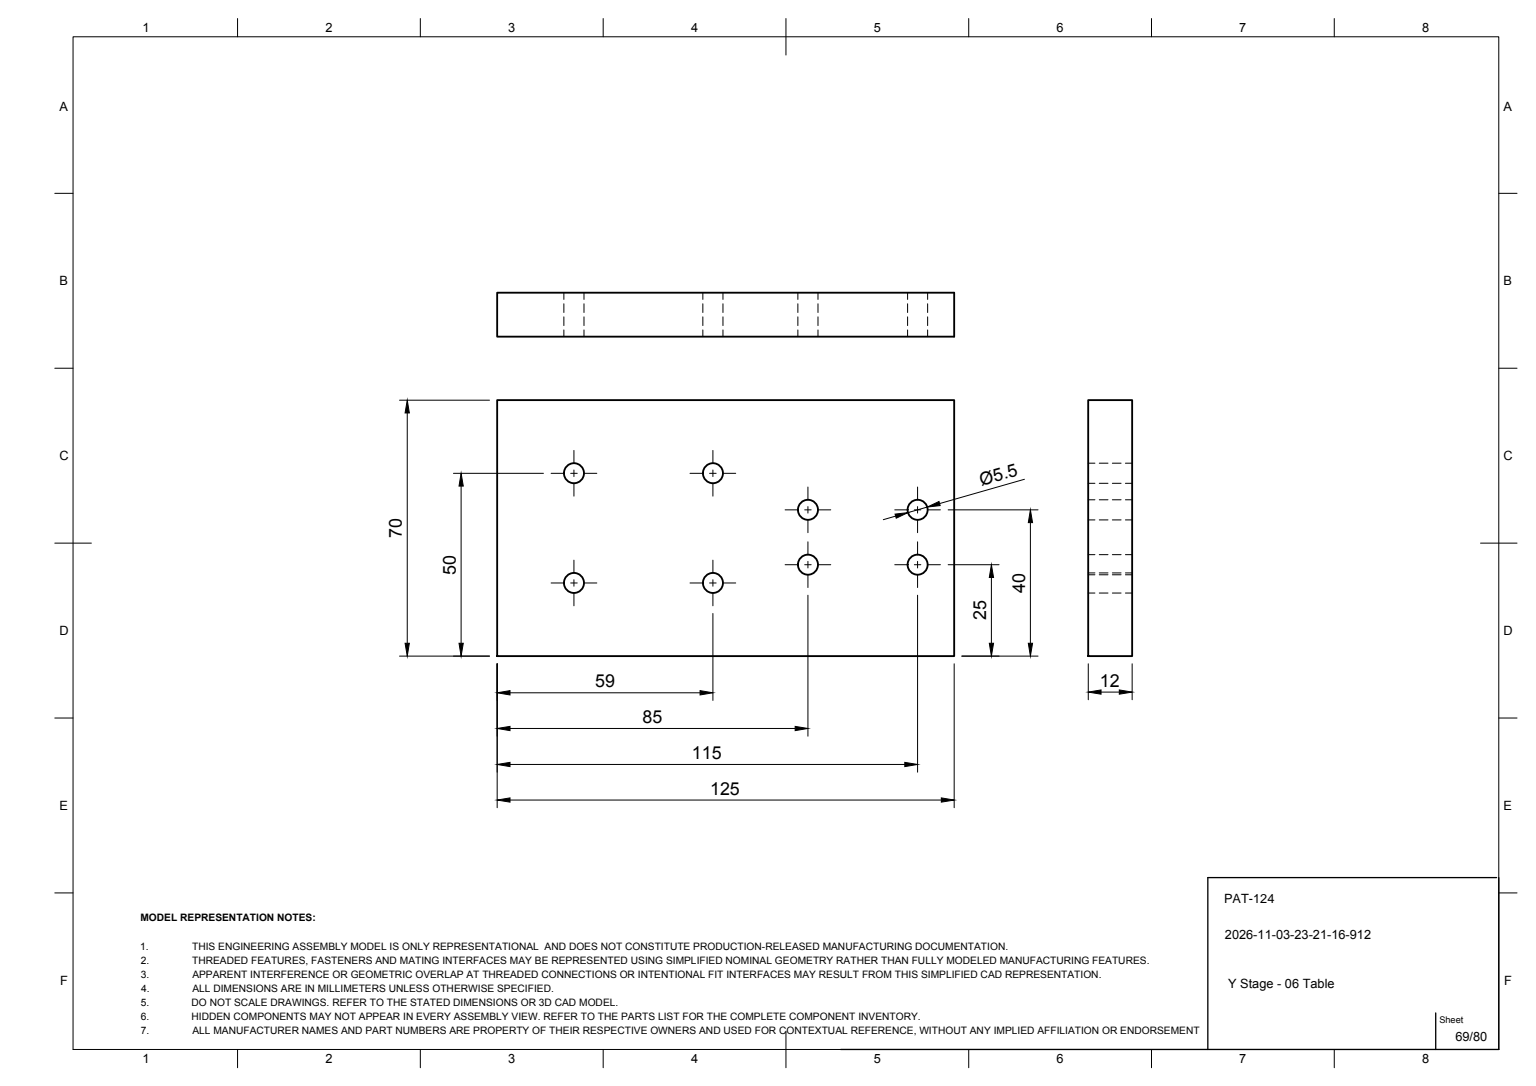
ISO-10303-21;
HEADER;
/* Generated by software containing ST-Developer
 * from STEP Tools, Inc. (www.steptools.com) 
 */

FILE_DESCRIPTION(
/* description */ ('XY cross-slide table'),
/* implementation_level */ '2;1');

FILE_NAME(
/* name */ 'Y Stage - 06 Table.step',
/* time_stamp */ '2026-10-28T03:22:46-07:00',
/* author */ (''),
/* organization */ (''),
/* preprocessor_version */ 'ST-DEVELOPER v20.2',
/* originating_system */ 'Autodesk Translation Framework v15.17.0.0',
/* authorisation */ '');

FILE_SCHEMA (('AUTOMOTIVE_DESIGN { 1 0 10303 214 3 1 1 }'));
ENDSEC;

DATA;
#10=MECHANICAL_DESIGN_GEOMETRIC_PRESENTATION_REPRESENTATION('',(#1763),#62984);
#1567=SHAPE_REPRESENTATION_RELATIONSHIP('SRR','None',#63425,#1650);
#1650=ADVANCED_BREP_SHAPE_REPRESENTATION('',(#1871),#62962);
#1763=STYLED_ITEM('',(#63905),#1871);
#1871=MANIFOLD_SOLID_BREP('Body1',#23062);
#2228=FACE_BOUND('',#5468,.T.);
#2229=FACE_BOUND('',#5469,.T.);
#2230=FACE_BOUND('',#5470,.T.);
#2231=FACE_BOUND('',#5471,.T.);
#2232=FACE_BOUND('',#5472,.T.);
#2233=FACE_BOUND('',#5473,.T.);
#2234=FACE_BOUND('',#5474,.T.);
#2235=FACE_BOUND('',#5475,.T.);
#2236=FACE_BOUND('',#5477,.T.);
#2237=FACE_BOUND('',#5478,.T.);
#2238=FACE_BOUND('',#5479,.T.);
#2239=FACE_BOUND('',#5480,.T.);
#2240=FACE_BOUND('',#5481,.T.);
#2241=FACE_BOUND('',#5482,.T.);
#2242=FACE_BOUND('',#5483,.T.);
#2243=FACE_BOUND('',#5484,.T.);
#2712=PLANE('',#25861);
#2713=PLANE('',#25862);
#2714=PLANE('',#25863);
#2715=PLANE('',#25864);
#2716=PLANE('',#25865);
#2717=PLANE('',#25866);
#3800=FACE_OUTER_BOUND('',#5455,.T.);
#3801=FACE_OUTER_BOUND('',#5456,.T.);
#3802=FACE_OUTER_BOUND('',#5457,.T.);
#3803=FACE_OUTER_BOUND('',#5458,.T.);
#3804=FACE_OUTER_BOUND('',#5459,.T.);
#3805=FACE_OUTER_BOUND('',#5460,.T.);
#3806=FACE_OUTER_BOUND('',#5461,.T.);
#3807=FACE_OUTER_BOUND('',#5462,.T.);
#3808=FACE_OUTER_BOUND('',#5463,.T.);
#3809=FACE_OUTER_BOUND('',#5464,.T.);
#3810=FACE_OUTER_BOUND('',#5465,.T.);
#3811=FACE_OUTER_BOUND('',#5466,.T.);
#3812=FACE_OUTER_BOUND('',#5467,.T.);
#3813=FACE_OUTER_BOUND('',#5476,.T.);
#5455=EDGE_LOOP('',(#19146,#19147,#19148,#19149));
#5456=EDGE_LOOP('',(#19150,#19151,#19152,#19153));
#5457=EDGE_LOOP('',(#19154,#19155,#19156,#19157));
#5458=EDGE_LOOP('',(#19158,#19159,#19160,#19161));
#5459=EDGE_LOOP('',(#19162,#19163,#19164,#19165));
#5460=EDGE_LOOP('',(#19166,#19167,#19168,#19169));
#5461=EDGE_LOOP('',(#19170,#19171,#19172,#19173));
#5462=EDGE_LOOP('',(#19174,#19175,#19176,#19177));
#5463=EDGE_LOOP('',(#19178,#19179,#19180,#19181));
#5464=EDGE_LOOP('',(#19182,#19183,#19184,#19185));
#5465=EDGE_LOOP('',(#19186,#19187,#19188,#19189));
#5466=EDGE_LOOP('',(#19190,#19191,#19192,#19193));
#5467=EDGE_LOOP('',(#19194,#19195,#19196,#19197));
#5468=EDGE_LOOP('',(#19198));
#5469=EDGE_LOOP('',(#19199));
#5470=EDGE_LOOP('',(#19200));
#5471=EDGE_LOOP('',(#19201));
#5472=EDGE_LOOP('',(#19202));
#5473=EDGE_LOOP('',(#19203));
#5474=EDGE_LOOP('',(#19204));
#5475=EDGE_LOOP('',(#19205));
#5476=EDGE_LOOP('',(#19206,#19207,#19208,#19209));
#5477=EDGE_LOOP('',(#19210));
#5478=EDGE_LOOP('',(#19211));
#5479=EDGE_LOOP('',(#19212));
#5480=EDGE_LOOP('',(#19213));
#5481=EDGE_LOOP('',(#19214));
#5482=EDGE_LOOP('',(#19215));
#5483=EDGE_LOOP('',(#19216));
#5484=EDGE_LOOP('',(#19217));
#6908=LINE('',#49767,#8395);
#6909=LINE('',#49773,#8396);
#6910=LINE('',#49779,#8397);
#6911=LINE('',#49785,#8398);
#6912=LINE('',#49791,#8399);
#6913=LINE('',#49797,#8400);
#6914=LINE('',#49803,#8401);
#6915=LINE('',#49809,#8402);
#6916=LINE('',#49814,#8403);
#6917=LINE('',#49816,#8404);
#6918=LINE('',#49818,#8405);
#6919=LINE('',#49819,#8406);
#6920=LINE('',#49822,#8407);
#6921=LINE('',#49824,#8408);
#6922=LINE('',#49825,#8409);
#6923=LINE('',#49828,#8410);
#6924=LINE('',#49830,#8411);
#6925=LINE('',#49831,#8412);
#6926=LINE('',#49833,#8413);
#6927=LINE('',#49834,#8414);
#8395=VECTOR('',#31141,0.275);
#8396=VECTOR('',#31148,0.275);
#8397=VECTOR('',#31155,0.275);
#8398=VECTOR('',#31162,0.275);
#8399=VECTOR('',#31169,0.275);
#8400=VECTOR('',#31176,0.275);
#8401=VECTOR('',#31183,0.275);
#8402=VECTOR('',#31190,0.275);
#8403=VECTOR('',#31195,1.);
#8404=VECTOR('',#31196,1.);
#8405=VECTOR('',#31197,1.);
#8406=VECTOR('',#31198,1.);
#8407=VECTOR('',#31201,1.);
#8408=VECTOR('',#31202,1.);
#8409=VECTOR('',#31203,1.);
#8410=VECTOR('',#31206,1.);
#8411=VECTOR('',#31207,1.);
#8412=VECTOR('',#31208,1.);
#8413=VECTOR('',#31211,1.);
#8414=VECTOR('',#31212,1.);
#9623=CIRCLE('',#25838,0.275);
#9624=CIRCLE('',#25839,0.275);
#9625=CIRCLE('',#25841,0.275);
#9626=CIRCLE('',#25842,0.275);
#9627=CIRCLE('',#25844,0.275);
#9628=CIRCLE('',#25845,0.275);
#9629=CIRCLE('',#25847,0.275);
#9630=CIRCLE('',#25848,0.275);
#9631=CIRCLE('',#25850,0.275);
#9632=CIRCLE('',#25851,0.275);
#9633=CIRCLE('',#25853,0.275);
#9634=CIRCLE('',#25854,0.275);
#9635=CIRCLE('',#25856,0.275);
#9636=CIRCLE('',#25857,0.275);
#9637=CIRCLE('',#25859,0.275);
#9638=CIRCLE('',#25860,0.275);
#11210=VERTEX_POINT('',#49764);
#11211=VERTEX_POINT('',#49766);
#11212=VERTEX_POINT('',#49770);
#11213=VERTEX_POINT('',#49772);
#11214=VERTEX_POINT('',#49776);
#11215=VERTEX_POINT('',#49778);
#11216=VERTEX_POINT('',#49782);
#11217=VERTEX_POINT('',#49784);
#11218=VERTEX_POINT('',#49788);
#11219=VERTEX_POINT('',#49790);
#11220=VERTEX_POINT('',#49794);
#11221=VERTEX_POINT('',#49796);
#11222=VERTEX_POINT('',#49800);
#11223=VERTEX_POINT('',#49802);
#11224=VERTEX_POINT('',#49806);
#11225=VERTEX_POINT('',#49808);
#11226=VERTEX_POINT('',#49812);
#11227=VERTEX_POINT('',#49813);
#11228=VERTEX_POINT('',#49815);
#11229=VERTEX_POINT('',#49817);
#11230=VERTEX_POINT('',#49821);
#11231=VERTEX_POINT('',#49823);
#11232=VERTEX_POINT('',#49827);
#11233=VERTEX_POINT('',#49829);
#13957=EDGE_CURVE('',#11210,#11210,#9623,.T.);
#13958=EDGE_CURVE('',#11210,#11211,#6908,.T.);
#13959=EDGE_CURVE('',#11211,#11211,#9624,.T.);
#13960=EDGE_CURVE('',#11212,#11212,#9625,.T.);
#13961=EDGE_CURVE('',#11212,#11213,#6909,.T.);
#13962=EDGE_CURVE('',#11213,#11213,#9626,.T.);
#13963=EDGE_CURVE('',#11214,#11214,#9627,.T.);
#13964=EDGE_CURVE('',#11214,#11215,#6910,.T.);
#13965=EDGE_CURVE('',#11215,#11215,#9628,.T.);
#13966=EDGE_CURVE('',#11216,#11216,#9629,.T.);
#13967=EDGE_CURVE('',#11216,#11217,#6911,.T.);
#13968=EDGE_CURVE('',#11217,#11217,#9630,.T.);
#13969=EDGE_CURVE('',#11218,#11218,#9631,.T.);
#13970=EDGE_CURVE('',#11218,#11219,#6912,.T.);
#13971=EDGE_CURVE('',#11219,#11219,#9632,.T.);
#13972=EDGE_CURVE('',#11220,#11220,#9633,.T.);
#13973=EDGE_CURVE('',#11220,#11221,#6913,.T.);
#13974=EDGE_CURVE('',#11221,#11221,#9634,.T.);
#13975=EDGE_CURVE('',#11222,#11222,#9635,.T.);
#13976=EDGE_CURVE('',#11222,#11223,#6914,.T.);
#13977=EDGE_CURVE('',#11223,#11223,#9636,.T.);
#13978=EDGE_CURVE('',#11224,#11224,#9637,.T.);
#13979=EDGE_CURVE('',#11224,#11225,#6915,.T.);
#13980=EDGE_CURVE('',#11225,#11225,#9638,.T.);
#13981=EDGE_CURVE('',#11226,#11227,#6916,.T.);
#13982=EDGE_CURVE('',#11227,#11228,#6917,.T.);
#13983=EDGE_CURVE('',#11229,#11228,#6918,.T.);
#13984=EDGE_CURVE('',#11226,#11229,#6919,.T.);
#13985=EDGE_CURVE('',#11230,#11226,#6920,.T.);
#13986=EDGE_CURVE('',#11231,#11229,#6921,.T.);
#13987=EDGE_CURVE('',#11230,#11231,#6922,.T.);
#13988=EDGE_CURVE('',#11232,#11230,#6923,.T.);
#13989=EDGE_CURVE('',#11233,#11231,#6924,.T.);
#13990=EDGE_CURVE('',#11232,#11233,#6925,.T.);
#13991=EDGE_CURVE('',#11227,#11232,#6926,.T.);
#13992=EDGE_CURVE('',#11228,#11233,#6927,.T.);
#19146=ORIENTED_EDGE('',*,*,#13957,.F.);
#19147=ORIENTED_EDGE('',*,*,#13958,.T.);
#19148=ORIENTED_EDGE('',*,*,#13959,.F.);
#19149=ORIENTED_EDGE('',*,*,#13958,.F.);
#19150=ORIENTED_EDGE('',*,*,#13960,.F.);
#19151=ORIENTED_EDGE('',*,*,#13961,.T.);
#19152=ORIENTED_EDGE('',*,*,#13962,.F.);
#19153=ORIENTED_EDGE('',*,*,#13961,.F.);
#19154=ORIENTED_EDGE('',*,*,#13963,.F.);
#19155=ORIENTED_EDGE('',*,*,#13964,.T.);
#19156=ORIENTED_EDGE('',*,*,#13965,.F.);
#19157=ORIENTED_EDGE('',*,*,#13964,.F.);
#19158=ORIENTED_EDGE('',*,*,#13966,.F.);
#19159=ORIENTED_EDGE('',*,*,#13967,.T.);
#19160=ORIENTED_EDGE('',*,*,#13968,.F.);
#19161=ORIENTED_EDGE('',*,*,#13967,.F.);
#19162=ORIENTED_EDGE('',*,*,#13969,.F.);
#19163=ORIENTED_EDGE('',*,*,#13970,.T.);
#19164=ORIENTED_EDGE('',*,*,#13971,.F.);
#19165=ORIENTED_EDGE('',*,*,#13970,.F.);
#19166=ORIENTED_EDGE('',*,*,#13972,.F.);
#19167=ORIENTED_EDGE('',*,*,#13973,.T.);
#19168=ORIENTED_EDGE('',*,*,#13974,.F.);
#19169=ORIENTED_EDGE('',*,*,#13973,.F.);
#19170=ORIENTED_EDGE('',*,*,#13975,.F.);
#19171=ORIENTED_EDGE('',*,*,#13976,.T.);
#19172=ORIENTED_EDGE('',*,*,#13977,.F.);
#19173=ORIENTED_EDGE('',*,*,#13976,.F.);
#19174=ORIENTED_EDGE('',*,*,#13978,.F.);
#19175=ORIENTED_EDGE('',*,*,#13979,.T.);
#19176=ORIENTED_EDGE('',*,*,#13980,.F.);
#19177=ORIENTED_EDGE('',*,*,#13979,.F.);
#19178=ORIENTED_EDGE('',*,*,#13981,.T.);
#19179=ORIENTED_EDGE('',*,*,#13982,.T.);
#19180=ORIENTED_EDGE('',*,*,#13983,.F.);
#19181=ORIENTED_EDGE('',*,*,#13984,.F.);
#19182=ORIENTED_EDGE('',*,*,#13985,.T.);
#19183=ORIENTED_EDGE('',*,*,#13984,.T.);
#19184=ORIENTED_EDGE('',*,*,#13986,.F.);
#19185=ORIENTED_EDGE('',*,*,#13987,.F.);
#19186=ORIENTED_EDGE('',*,*,#13988,.T.);
#19187=ORIENTED_EDGE('',*,*,#13987,.T.);
#19188=ORIENTED_EDGE('',*,*,#13989,.F.);
#19189=ORIENTED_EDGE('',*,*,#13990,.F.);
#19190=ORIENTED_EDGE('',*,*,#13991,.T.);
#19191=ORIENTED_EDGE('',*,*,#13990,.T.);
#19192=ORIENTED_EDGE('',*,*,#13992,.F.);
#19193=ORIENTED_EDGE('',*,*,#13982,.F.);
#19194=ORIENTED_EDGE('',*,*,#13992,.T.);
#19195=ORIENTED_EDGE('',*,*,#13989,.T.);
#19196=ORIENTED_EDGE('',*,*,#13986,.T.);
#19197=ORIENTED_EDGE('',*,*,#13983,.T.);
#19198=ORIENTED_EDGE('',*,*,#13980,.T.);
#19199=ORIENTED_EDGE('',*,*,#13977,.T.);
#19200=ORIENTED_EDGE('',*,*,#13974,.T.);
#19201=ORIENTED_EDGE('',*,*,#13971,.T.);
#19202=ORIENTED_EDGE('',*,*,#13968,.T.);
#19203=ORIENTED_EDGE('',*,*,#13965,.T.);
#19204=ORIENTED_EDGE('',*,*,#13962,.T.);
#19205=ORIENTED_EDGE('',*,*,#13959,.T.);
#19206=ORIENTED_EDGE('',*,*,#13991,.F.);
#19207=ORIENTED_EDGE('',*,*,#13981,.F.);
#19208=ORIENTED_EDGE('',*,*,#13985,.F.);
#19209=ORIENTED_EDGE('',*,*,#13988,.F.);
#19210=ORIENTED_EDGE('',*,*,#13978,.T.);
#19211=ORIENTED_EDGE('',*,*,#13975,.T.);
#19212=ORIENTED_EDGE('',*,*,#13972,.T.);
#19213=ORIENTED_EDGE('',*,*,#13969,.T.);
#19214=ORIENTED_EDGE('',*,*,#13966,.T.);
#19215=ORIENTED_EDGE('',*,*,#13963,.T.);
#19216=ORIENTED_EDGE('',*,*,#13960,.T.);
#19217=ORIENTED_EDGE('',*,*,#13957,.T.);
#21446=CYLINDRICAL_SURFACE('',#25837,0.275);
#21447=CYLINDRICAL_SURFACE('',#25840,0.275);
#21448=CYLINDRICAL_SURFACE('',#25843,0.275);
#21449=CYLINDRICAL_SURFACE('',#25846,0.275);
#21450=CYLINDRICAL_SURFACE('',#25849,0.275);
#21451=CYLINDRICAL_SURFACE('',#25852,0.275);
#21452=CYLINDRICAL_SURFACE('',#25855,0.275);
#21453=CYLINDRICAL_SURFACE('',#25858,0.275);
#22581=ADVANCED_FACE('',(#3800),#21446,.F.);
#22582=ADVANCED_FACE('',(#3801),#21447,.F.);
#22583=ADVANCED_FACE('',(#3802),#21448,.F.);
#22584=ADVANCED_FACE('',(#3803),#21449,.F.);
#22585=ADVANCED_FACE('',(#3804),#21450,.F.);
#22586=ADVANCED_FACE('',(#3805),#21451,.F.);
#22587=ADVANCED_FACE('',(#3806),#21452,.F.);
#22588=ADVANCED_FACE('',(#3807),#21453,.F.);
#22589=ADVANCED_FACE('',(#3808),#2712,.T.);
#22590=ADVANCED_FACE('',(#3809),#2713,.T.);
#22591=ADVANCED_FACE('',(#3810),#2714,.T.);
#22592=ADVANCED_FACE('',(#3811),#2715,.T.);
#22593=ADVANCED_FACE('',(#3812,#2228,#2229,#2230,#2231,#2232,#2233,#2234,
#2235),#2716,.T.);
#22594=ADVANCED_FACE('',(#3813,#2236,#2237,#2238,#2239,#2240,#2241,#2242,
#2243),#2717,.F.);
#23062=CLOSED_SHELL('',(#22581,#22582,#22583,#22584,#22585,#22586,#22587,
#22588,#22589,#22590,#22591,#22592,#22593,#22594));
#25836=AXIS2_PLACEMENT_3D('',#49762,#31135,#31136);
#25837=AXIS2_PLACEMENT_3D('',#49763,#31137,#31138);
#25838=AXIS2_PLACEMENT_3D('',#49765,#31139,#31140);
#25839=AXIS2_PLACEMENT_3D('',#49768,#31142,#31143);
#25840=AXIS2_PLACEMENT_3D('',#49769,#31144,#31145);
#25841=AXIS2_PLACEMENT_3D('',#49771,#31146,#31147);
#25842=AXIS2_PLACEMENT_3D('',#49774,#31149,#31150);
#25843=AXIS2_PLACEMENT_3D('',#49775,#31151,#31152);
#25844=AXIS2_PLACEMENT_3D('',#49777,#31153,#31154);
#25845=AXIS2_PLACEMENT_3D('',#49780,#31156,#31157);
#25846=AXIS2_PLACEMENT_3D('',#49781,#31158,#31159);
#25847=AXIS2_PLACEMENT_3D('',#49783,#31160,#31161);
#25848=AXIS2_PLACEMENT_3D('',#49786,#31163,#31164);
#25849=AXIS2_PLACEMENT_3D('',#49787,#31165,#31166);
#25850=AXIS2_PLACEMENT_3D('',#49789,#31167,#31168);
#25851=AXIS2_PLACEMENT_3D('',#49792,#31170,#31171);
#25852=AXIS2_PLACEMENT_3D('',#49793,#31172,#31173);
#25853=AXIS2_PLACEMENT_3D('',#49795,#31174,#31175);
#25854=AXIS2_PLACEMENT_3D('',#49798,#31177,#31178);
#25855=AXIS2_PLACEMENT_3D('',#49799,#31179,#31180);
#25856=AXIS2_PLACEMENT_3D('',#49801,#31181,#31182);
#25857=AXIS2_PLACEMENT_3D('',#49804,#31184,#31185);
#25858=AXIS2_PLACEMENT_3D('',#49805,#31186,#31187);
#25859=AXIS2_PLACEMENT_3D('',#49807,#31188,#31189);
#25860=AXIS2_PLACEMENT_3D('',#49810,#31191,#31192);
#25861=AXIS2_PLACEMENT_3D('',#49811,#31193,#31194);
#25862=AXIS2_PLACEMENT_3D('',#49820,#31199,#31200);
#25863=AXIS2_PLACEMENT_3D('',#49826,#31204,#31205);
#25864=AXIS2_PLACEMENT_3D('',#49832,#31209,#31210);
#25865=AXIS2_PLACEMENT_3D('',#49835,#31213,#31214);
#25866=AXIS2_PLACEMENT_3D('',#49836,#31215,#31216);
#31135=DIRECTION('axis',(0.,0.,1.));
#31136=DIRECTION('refdir',(1.,0.,0.));
#31137=DIRECTION('center_axis',(0.,0.,1.));
#31138=DIRECTION('ref_axis',(1.,0.,0.));
#31139=DIRECTION('center_axis',(0.,0.,1.));
#31140=DIRECTION('ref_axis',(1.,0.,0.));
#31141=DIRECTION('',(0.,0.,1.));
#31142=DIRECTION('center_axis',(0.,0.,-1.));
#31143=DIRECTION('ref_axis',(1.,0.,0.));
#31144=DIRECTION('center_axis',(0.,0.,1.));
#31145=DIRECTION('ref_axis',(1.,0.,0.));
#31146=DIRECTION('center_axis',(0.,0.,1.));
#31147=DIRECTION('ref_axis',(1.,0.,0.));
#31148=DIRECTION('',(0.,0.,1.));
#31149=DIRECTION('center_axis',(0.,0.,-1.));
#31150=DIRECTION('ref_axis',(1.,0.,0.));
#31151=DIRECTION('center_axis',(0.,0.,1.));
#31152=DIRECTION('ref_axis',(1.,0.,0.));
#31153=DIRECTION('center_axis',(0.,0.,1.));
#31154=DIRECTION('ref_axis',(1.,0.,0.));
#31155=DIRECTION('',(0.,0.,1.));
#31156=DIRECTION('center_axis',(0.,0.,-1.));
#31157=DIRECTION('ref_axis',(1.,0.,0.));
#31158=DIRECTION('center_axis',(0.,0.,1.));
#31159=DIRECTION('ref_axis',(1.,0.,0.));
#31160=DIRECTION('center_axis',(0.,0.,1.));
#31161=DIRECTION('ref_axis',(1.,0.,0.));
#31162=DIRECTION('',(0.,0.,1.));
#31163=DIRECTION('center_axis',(0.,0.,-1.));
#31164=DIRECTION('ref_axis',(1.,0.,0.));
#31165=DIRECTION('center_axis',(0.,0.,1.));
#31166=DIRECTION('ref_axis',(1.,0.,0.));
#31167=DIRECTION('center_axis',(0.,0.,1.));
#31168=DIRECTION('ref_axis',(1.,0.,0.));
#31169=DIRECTION('',(0.,0.,1.));
#31170=DIRECTION('center_axis',(0.,0.,-1.));
#31171=DIRECTION('ref_axis',(1.,0.,0.));
#31172=DIRECTION('center_axis',(0.,0.,1.));
#31173=DIRECTION('ref_axis',(1.,0.,0.));
#31174=DIRECTION('center_axis',(0.,0.,1.));
#31175=DIRECTION('ref_axis',(1.,0.,0.));
#31176=DIRECTION('',(0.,0.,1.));
#31177=DIRECTION('center_axis',(0.,0.,-1.));
#31178=DIRECTION('ref_axis',(1.,0.,0.));
#31179=DIRECTION('center_axis',(0.,0.,1.));
#31180=DIRECTION('ref_axis',(1.,0.,0.));
#31181=DIRECTION('center_axis',(0.,0.,1.));
#31182=DIRECTION('ref_axis',(1.,0.,0.));
#31183=DIRECTION('',(0.,0.,1.));
#31184=DIRECTION('center_axis',(0.,0.,-1.));
#31185=DIRECTION('ref_axis',(1.,0.,0.));
#31186=DIRECTION('center_axis',(0.,0.,1.));
#31187=DIRECTION('ref_axis',(1.,0.,0.));
#31188=DIRECTION('center_axis',(0.,0.,1.));
#31189=DIRECTION('ref_axis',(1.,0.,0.));
#31190=DIRECTION('',(0.,0.,1.));
#31191=DIRECTION('center_axis',(0.,0.,-1.));
#31192=DIRECTION('ref_axis',(1.,0.,0.));
#31193=DIRECTION('center_axis',(0.,1.,0.));
#31194=DIRECTION('ref_axis',(-1.,0.,0.));
#31195=DIRECTION('',(-1.,0.,0.));
#31196=DIRECTION('',(0.,0.,1.));
#31197=DIRECTION('',(-1.,0.,0.));
#31198=DIRECTION('',(0.,0.,1.));
#31199=DIRECTION('center_axis',(1.,0.,0.));
#31200=DIRECTION('ref_axis',(0.,1.,0.));
#31201=DIRECTION('',(0.,1.,0.));
#31202=DIRECTION('',(0.,1.,0.));
#31203=DIRECTION('',(0.,0.,1.));
#31204=DIRECTION('center_axis',(0.,-1.,0.));
#31205=DIRECTION('ref_axis',(1.,0.,0.));
#31206=DIRECTION('',(1.,0.,0.));
#31207=DIRECTION('',(1.,0.,0.));
#31208=DIRECTION('',(0.,0.,1.));
#31209=DIRECTION('center_axis',(-1.,0.,0.));
#31210=DIRECTION('ref_axis',(0.,-1.,0.));
#31211=DIRECTION('',(0.,-1.,0.));
#31212=DIRECTION('',(0.,-1.,0.));
#31213=DIRECTION('center_axis',(0.,0.,1.));
#31214=DIRECTION('ref_axis',(1.,0.,0.));
#31215=DIRECTION('center_axis',(0.,0.,1.));
#31216=DIRECTION('ref_axis',(1.,0.,0.));
#49762=CARTESIAN_POINT('',(0.,0.,0.));
#49763=CARTESIAN_POINT('Origin',(14.,-1.5,5.9));
#49764=CARTESIAN_POINT('',(13.725,-1.5,6.));
#49765=CARTESIAN_POINT('Origin',(14.,-1.5,6.));
#49766=CARTESIAN_POINT('',(13.725,-1.5,7.2));
#49767=CARTESIAN_POINT('',(13.725,-1.5,5.9));
#49768=CARTESIAN_POINT('Origin',(14.,-1.5,7.2));
#49769=CARTESIAN_POINT('Origin',(12.5,1.5,5.9));
#49770=CARTESIAN_POINT('',(12.225,1.5,6.));
#49771=CARTESIAN_POINT('Origin',(12.5,1.5,6.));
#49772=CARTESIAN_POINT('',(12.225,1.5,7.2));
#49773=CARTESIAN_POINT('',(12.225,1.5,5.9));
#49774=CARTESIAN_POINT('Origin',(12.5,1.5,7.2));
#49775=CARTESIAN_POINT('Origin',(12.5,-1.5,5.9));
#49776=CARTESIAN_POINT('',(12.225,-1.5,6.));
#49777=CARTESIAN_POINT('Origin',(12.5,-1.5,6.));
#49778=CARTESIAN_POINT('',(12.225,-1.5,7.2));
#49779=CARTESIAN_POINT('',(12.225,-1.5,5.9));
#49780=CARTESIAN_POINT('Origin',(12.5,-1.5,7.2));
#49781=CARTESIAN_POINT('Origin',(14.,1.5,5.9));
#49782=CARTESIAN_POINT('',(13.725,1.5,6.));
#49783=CARTESIAN_POINT('Origin',(14.,1.5,6.));
#49784=CARTESIAN_POINT('',(13.725,1.5,7.2));
#49785=CARTESIAN_POINT('',(13.725,1.5,5.9));
#49786=CARTESIAN_POINT('Origin',(14.,1.5,7.2));
#49787=CARTESIAN_POINT('Origin',(15.,-7.9,5.1));
#49788=CARTESIAN_POINT('',(14.725,-7.9,6.));
#49789=CARTESIAN_POINT('Origin',(15.,-7.9,6.));
#49790=CARTESIAN_POINT('',(14.725,-7.9,7.2));
#49791=CARTESIAN_POINT('',(14.725,-7.9,5.1));
#49792=CARTESIAN_POINT('Origin',(15.,-7.9,7.2));
#49793=CARTESIAN_POINT('Origin',(12.,-4.1,5.1));
#49794=CARTESIAN_POINT('',(11.725,-4.1,6.));
#49795=CARTESIAN_POINT('Origin',(12.,-4.1,6.));
#49796=CARTESIAN_POINT('',(11.725,-4.1,7.2));
#49797=CARTESIAN_POINT('',(11.725,-4.1,5.1));
#49798=CARTESIAN_POINT('Origin',(12.,-4.1,7.2));
#49799=CARTESIAN_POINT('Origin',(12.,-7.9,5.1));
#49800=CARTESIAN_POINT('',(11.725,-7.9,6.));
#49801=CARTESIAN_POINT('Origin',(12.,-7.9,6.));
#49802=CARTESIAN_POINT('',(11.725,-7.9,7.2));
#49803=CARTESIAN_POINT('',(11.725,-7.9,5.1));
#49804=CARTESIAN_POINT('Origin',(12.,-7.9,7.2));
#49805=CARTESIAN_POINT('Origin',(15.,-4.1,5.1));
#49806=CARTESIAN_POINT('',(14.725,-4.1,6.));
#49807=CARTESIAN_POINT('Origin',(15.,-4.1,6.));
#49808=CARTESIAN_POINT('',(14.725,-4.1,7.2));
#49809=CARTESIAN_POINT('',(14.725,-4.1,5.1));
#49810=CARTESIAN_POINT('Origin',(15.,-4.1,7.2));
#49811=CARTESIAN_POINT('Origin',(17.,2.5,6.));
#49812=CARTESIAN_POINT('',(17.,2.5,6.));
#49813=CARTESIAN_POINT('',(10.,2.5,6.));
#49814=CARTESIAN_POINT('',(17.,2.5,6.));
#49815=CARTESIAN_POINT('',(10.,2.5,7.2));
#49816=CARTESIAN_POINT('',(10.,2.5,6.));
#49817=CARTESIAN_POINT('',(17.,2.5,7.2));
#49818=CARTESIAN_POINT('',(17.,2.5,7.2));
#49819=CARTESIAN_POINT('',(17.,2.5,6.));
#49820=CARTESIAN_POINT('Origin',(17.,-10.,6.));
#49821=CARTESIAN_POINT('',(17.,-10.,6.));
#49822=CARTESIAN_POINT('',(17.,-10.,6.));
#49823=CARTESIAN_POINT('',(17.,-10.,7.2));
#49824=CARTESIAN_POINT('',(17.,-10.,7.2));
#49825=CARTESIAN_POINT('',(17.,-10.,6.));
#49826=CARTESIAN_POINT('Origin',(10.,-10.,6.));
#49827=CARTESIAN_POINT('',(10.,-10.,6.));
#49828=CARTESIAN_POINT('',(10.,-10.,6.));
#49829=CARTESIAN_POINT('',(10.,-10.,7.2));
#49830=CARTESIAN_POINT('',(10.,-10.,7.2));
#49831=CARTESIAN_POINT('',(10.,-10.,6.));
#49832=CARTESIAN_POINT('Origin',(10.,2.5,6.));
#49833=CARTESIAN_POINT('',(10.,2.5,6.));
#49834=CARTESIAN_POINT('',(10.,2.5,7.2));
#49835=CARTESIAN_POINT('Origin',(13.5,-3.75,7.2));
#49836=CARTESIAN_POINT('Origin',(13.5,-3.75,6.));
#62863=UNCERTAINTY_MEASURE_WITH_UNIT(LENGTH_MEASURE(0.001),#62985,
'DISTANCE_ACCURACY_VALUE',
'Maximum model space distance between geometric entities at asserted c
onnectivities');
#62885=UNCERTAINTY_MEASURE_WITH_UNIT(LENGTH_MEASURE(0.001),#62985,
'DISTANCE_ACCURACY_VALUE',
'Maximum model space distance between geometric entities at asserted c
onnectivities');
#62962=(
GEOMETRIC_REPRESENTATION_CONTEXT(3)
GLOBAL_UNCERTAINTY_ASSIGNED_CONTEXT((#62863))
GLOBAL_UNIT_ASSIGNED_CONTEXT((#62985,#62987,#62988))
REPRESENTATION_CONTEXT('','3D')
);
#62984=(
GEOMETRIC_REPRESENTATION_CONTEXT(3)
GLOBAL_UNCERTAINTY_ASSIGNED_CONTEXT((#62885))
GLOBAL_UNIT_ASSIGNED_CONTEXT((#62985,#62987,#62988))
REPRESENTATION_CONTEXT('','3D')
);
#62985=(
LENGTH_UNIT()
NAMED_UNIT(*)
SI_UNIT(.CENTI.,.METRE.)
);
#62987=(
NAMED_UNIT(*)
PLANE_ANGLE_UNIT()
SI_UNIT($,.RADIAN.)
);
#62988=(
NAMED_UNIT(*)
SI_UNIT($,.STERADIAN.)
SOLID_ANGLE_UNIT()
);
#63065=SHAPE_DEFINITION_REPRESENTATION(#63253,#63425);
#63253=PRODUCT_DEFINITION_SHAPE('',$,#63524);
#63425=SHAPE_REPRESENTATION('',(#25836),#62962);
#63447=PRODUCT_DEFINITION_CONTEXT('part definition',#63743,'design');
#63524=PRODUCT_DEFINITION('Y Stage - 06 Table','Y Stage - 06 Table',#63622,
#63447);
#63622=PRODUCT_DEFINITION_FORMATION('',$,#63821);
#63743=APPLICATION_CONTEXT(
'Core Data for Automotive Mechanical Design Process');
#63744=PRODUCT_CONTEXT('part definition',#63743,'mechanical');
#63821=PRODUCT('Y Stage - 06 Table','Y Stage - 06 Table',
'Y Stage - 06 Table',(#63744));
#63899=COLOUR_RGB('Sky Blue',0.24,0.69,0.87);
#63900=FILL_AREA_STYLE_COLOUR('',#63899);
#63901=FILL_AREA_STYLE('',(#63900));
#63902=SURFACE_STYLE_FILL_AREA(#63901);
#63903=SURFACE_SIDE_STYLE('',(#63902));
#63904=SURFACE_STYLE_USAGE(.BOTH.,#63903);
#63905=PRESENTATION_STYLE_ASSIGNMENT((#63904));
ENDSEC;
END-ISO-10303-21;
